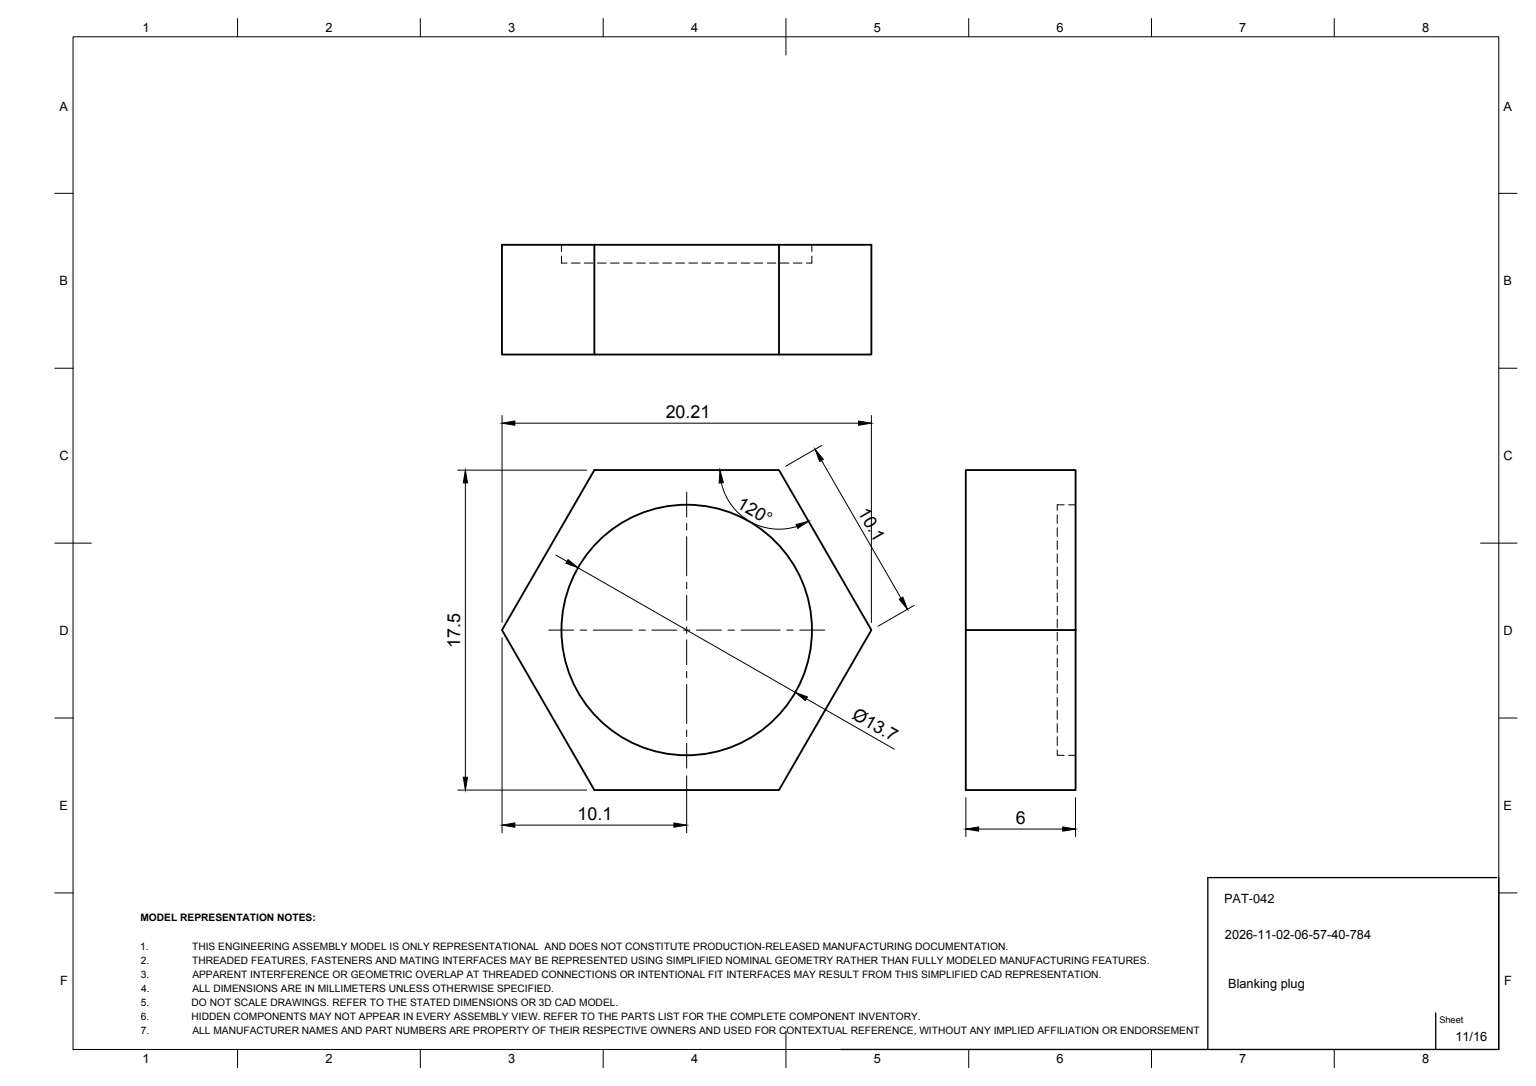
ISO-10303-21;
HEADER;
/* Generated by software containing ST-Developer
 * from STEP Tools, Inc. (www.steptools.com) 
 */

FILE_DESCRIPTION(
/* description */ ('Manifold and mounting hardware'),
/* implementation_level */ '2;1');

FILE_NAME(
/* name */ 'Blanking plug.step',
/* time_stamp */ '2026-10-28T21:46:49-07:00',
/* author */ (''),
/* organization */ (''),
/* preprocessor_version */ 'ST-DEVELOPER v20.2',
/* originating_system */ 'Autodesk Translation Framework v15.17.0.0',
/* authorisation */ '');

FILE_SCHEMA (('AUTOMOTIVE_DESIGN { 1 0 10303 214 3 1 1 }'));
ENDSEC;

DATA;
#10=MECHANICAL_DESIGN_GEOMETRIC_PRESENTATION_REPRESENTATION('',(#158),#5638);
#130=SHAPE_REPRESENTATION_RELATIONSHIP('SRR','None',#5709,#144);
#144=ADVANCED_BREP_SHAPE_REPRESENTATION('',(#172),#5631);
#158=STYLED_ITEM('',(#5874),#172);
#172=MANIFOLD_SOLID_BREP('Body1',#3148);
#240=FACE_BOUND('',#714,.T.);
#317=CYLINDRICAL_SURFACE('',#3559,0.685);
#463=FACE_OUTER_BOUND('',#711,.T.);
#464=FACE_OUTER_BOUND('',#712,.T.);
#465=FACE_OUTER_BOUND('',#713,.T.);
#466=FACE_OUTER_BOUND('',#715,.T.);
#467=FACE_OUTER_BOUND('',#716,.T.);
#468=FACE_OUTER_BOUND('',#717,.T.);
#469=FACE_OUTER_BOUND('',#718,.T.);
#470=FACE_OUTER_BOUND('',#719,.T.);
#471=FACE_OUTER_BOUND('',#720,.T.);
#472=FACE_OUTER_BOUND('',#721,.T.);
#711=EDGE_LOOP('',(#2632,#2633,#2634,#2635));
#712=EDGE_LOOP('',(#2636));
#713=EDGE_LOOP('',(#2637,#2638,#2639,#2640,#2641,#2642));
#714=EDGE_LOOP('',(#2643));
#715=EDGE_LOOP('',(#2644,#2645,#2646,#2647));
#716=EDGE_LOOP('',(#2648,#2649,#2650,#2651));
#717=EDGE_LOOP('',(#2652,#2653,#2654,#2655));
#718=EDGE_LOOP('',(#2656,#2657,#2658,#2659));
#719=EDGE_LOOP('',(#2660,#2661,#2662,#2663));
#720=EDGE_LOOP('',(#2664,#2665,#2666,#2667));
#721=EDGE_LOOP('',(#2668,#2669,#2670,#2671,#2672,#2673));
#868=CIRCLE('',#3560,0.685);
#869=CIRCLE('',#3561,0.685);
#1080=LINE('',#5349,#1327);
#1081=LINE('',#5355,#1328);
#1082=LINE('',#5357,#1329);
#1083=LINE('',#5359,#1330);
#1084=LINE('',#5361,#1331);
#1085=LINE('',#5363,#1332);
#1086=LINE('',#5364,#1333);
#1087=LINE('',#5367,#1334);
#1088=LINE('',#5369,#1335);
#1089=LINE('',#5370,#1336);
#1090=LINE('',#5373,#1337);
#1091=LINE('',#5374,#1338);
#1092=LINE('',#5377,#1339);
#1093=LINE('',#5378,#1340);
#1094=LINE('',#5381,#1341);
#1095=LINE('',#5382,#1342);
#1096=LINE('',#5385,#1343);
#1097=LINE('',#5386,#1344);
#1098=LINE('',#5388,#1345);
#1327=VECTOR('',#4359,0.685);
#1328=VECTOR('',#4366,1.);
#1329=VECTOR('',#4367,1.);
#1330=VECTOR('',#4368,1.);
#1331=VECTOR('',#4369,1.);
#1332=VECTOR('',#4370,1.);
#1333=VECTOR('',#4371,1.);
#1334=VECTOR('',#4374,1.);
#1335=VECTOR('',#4375,1.);
#1336=VECTOR('',#4376,1.);
#1337=VECTOR('',#4379,1.);
#1338=VECTOR('',#4380,1.);
#1339=VECTOR('',#4383,1.);
#1340=VECTOR('',#4384,1.);
#1341=VECTOR('',#4387,1.);
#1342=VECTOR('',#4388,1.);
#1343=VECTOR('',#4391,1.);
#1344=VECTOR('',#4392,1.);
#1345=VECTOR('',#4395,1.);
#1586=VERTEX_POINT('',#5346);
#1587=VERTEX_POINT('',#5348);
#1588=VERTEX_POINT('',#5353);
#1589=VERTEX_POINT('',#5354);
#1590=VERTEX_POINT('',#5356);
#1591=VERTEX_POINT('',#5358);
#1592=VERTEX_POINT('',#5360);
#1593=VERTEX_POINT('',#5362);
#1594=VERTEX_POINT('',#5366);
#1595=VERTEX_POINT('',#5368);
#1596=VERTEX_POINT('',#5372);
#1597=VERTEX_POINT('',#5376);
#1598=VERTEX_POINT('',#5380);
#1599=VERTEX_POINT('',#5384);
#1945=EDGE_CURVE('',#1586,#1586,#868,.T.);
#1946=EDGE_CURVE('',#1586,#1587,#1080,.T.);
#1947=EDGE_CURVE('',#1587,#1587,#869,.T.);
#1948=EDGE_CURVE('',#1588,#1589,#1081,.T.);
#1949=EDGE_CURVE('',#1590,#1588,#1082,.T.);
#1950=EDGE_CURVE('',#1591,#1590,#1083,.T.);
#1951=EDGE_CURVE('',#1592,#1591,#1084,.T.);
#1952=EDGE_CURVE('',#1593,#1592,#1085,.T.);
#1953=EDGE_CURVE('',#1589,#1593,#1086,.T.);
#1954=EDGE_CURVE('',#1588,#1594,#1087,.T.);
#1955=EDGE_CURVE('',#1595,#1594,#1088,.T.);
#1956=EDGE_CURVE('',#1590,#1595,#1089,.T.);
#1957=EDGE_CURVE('',#1596,#1595,#1090,.T.);
#1958=EDGE_CURVE('',#1591,#1596,#1091,.T.);
#1959=EDGE_CURVE('',#1597,#1596,#1092,.T.);
#1960=EDGE_CURVE('',#1592,#1597,#1093,.T.);
#1961=EDGE_CURVE('',#1598,#1597,#1094,.T.);
#1962=EDGE_CURVE('',#1593,#1598,#1095,.T.);
#1963=EDGE_CURVE('',#1599,#1598,#1096,.T.);
#1964=EDGE_CURVE('',#1589,#1599,#1097,.T.);
#1965=EDGE_CURVE('',#1594,#1599,#1098,.T.);
#2632=ORIENTED_EDGE('',*,*,#1945,.F.);
#2633=ORIENTED_EDGE('',*,*,#1946,.T.);
#2634=ORIENTED_EDGE('',*,*,#1947,.T.);
#2635=ORIENTED_EDGE('',*,*,#1946,.F.);
#2636=ORIENTED_EDGE('',*,*,#1947,.F.);
#2637=ORIENTED_EDGE('',*,*,#1948,.F.);
#2638=ORIENTED_EDGE('',*,*,#1949,.F.);
#2639=ORIENTED_EDGE('',*,*,#1950,.F.);
#2640=ORIENTED_EDGE('',*,*,#1951,.F.);
#2641=ORIENTED_EDGE('',*,*,#1952,.F.);
#2642=ORIENTED_EDGE('',*,*,#1953,.F.);
#2643=ORIENTED_EDGE('',*,*,#1945,.T.);
#2644=ORIENTED_EDGE('',*,*,#1949,.T.);
#2645=ORIENTED_EDGE('',*,*,#1954,.T.);
#2646=ORIENTED_EDGE('',*,*,#1955,.F.);
#2647=ORIENTED_EDGE('',*,*,#1956,.F.);
#2648=ORIENTED_EDGE('',*,*,#1950,.T.);
#2649=ORIENTED_EDGE('',*,*,#1956,.T.);
#2650=ORIENTED_EDGE('',*,*,#1957,.F.);
#2651=ORIENTED_EDGE('',*,*,#1958,.F.);
#2652=ORIENTED_EDGE('',*,*,#1951,.T.);
#2653=ORIENTED_EDGE('',*,*,#1958,.T.);
#2654=ORIENTED_EDGE('',*,*,#1959,.F.);
#2655=ORIENTED_EDGE('',*,*,#1960,.F.);
#2656=ORIENTED_EDGE('',*,*,#1952,.T.);
#2657=ORIENTED_EDGE('',*,*,#1960,.T.);
#2658=ORIENTED_EDGE('',*,*,#1961,.F.);
#2659=ORIENTED_EDGE('',*,*,#1962,.F.);
#2660=ORIENTED_EDGE('',*,*,#1953,.T.);
#2661=ORIENTED_EDGE('',*,*,#1962,.T.);
#2662=ORIENTED_EDGE('',*,*,#1963,.F.);
#2663=ORIENTED_EDGE('',*,*,#1964,.F.);
#2664=ORIENTED_EDGE('',*,*,#1948,.T.);
#2665=ORIENTED_EDGE('',*,*,#1964,.T.);
#2666=ORIENTED_EDGE('',*,*,#1965,.F.);
#2667=ORIENTED_EDGE('',*,*,#1954,.F.);
#2668=ORIENTED_EDGE('',*,*,#1965,.T.);
#2669=ORIENTED_EDGE('',*,*,#1963,.T.);
#2670=ORIENTED_EDGE('',*,*,#1961,.T.);
#2671=ORIENTED_EDGE('',*,*,#1959,.T.);
#2672=ORIENTED_EDGE('',*,*,#1957,.T.);
#2673=ORIENTED_EDGE('',*,*,#1955,.T.);
#2918=PLANE('',#3562);
#2919=PLANE('',#3563);
#2920=PLANE('',#3564);
#2921=PLANE('',#3565);
#2922=PLANE('',#3566);
#2923=PLANE('',#3567);
#2924=PLANE('',#3568);
#2925=PLANE('',#3569);
#2926=PLANE('',#3570);
#3087=ADVANCED_FACE('',(#463),#317,.F.);
#3088=ADVANCED_FACE('',(#464),#2918,.F.);
#3089=ADVANCED_FACE('',(#465,#240),#2919,.F.);
#3090=ADVANCED_FACE('',(#466),#2920,.T.);
#3091=ADVANCED_FACE('',(#467),#2921,.T.);
#3092=ADVANCED_FACE('',(#468),#2922,.T.);
#3093=ADVANCED_FACE('',(#469),#2923,.T.);
#3094=ADVANCED_FACE('',(#470),#2924,.T.);
#3095=ADVANCED_FACE('',(#471),#2925,.T.);
#3096=ADVANCED_FACE('',(#472),#2926,.T.);
#3148=CLOSED_SHELL('',(#3087,#3088,#3089,#3090,#3091,#3092,#3093,#3094,
#3095,#3096));
#3558=AXIS2_PLACEMENT_3D('',#5344,#4353,#4354);
#3559=AXIS2_PLACEMENT_3D('',#5345,#4355,#4356);
#3560=AXIS2_PLACEMENT_3D('',#5347,#4357,#4358);
#3561=AXIS2_PLACEMENT_3D('',#5350,#4360,#4361);
#3562=AXIS2_PLACEMENT_3D('',#5351,#4362,#4363);
#3563=AXIS2_PLACEMENT_3D('',#5352,#4364,#4365);
#3564=AXIS2_PLACEMENT_3D('',#5365,#4372,#4373);
#3565=AXIS2_PLACEMENT_3D('',#5371,#4377,#4378);
#3566=AXIS2_PLACEMENT_3D('',#5375,#4381,#4382);
#3567=AXIS2_PLACEMENT_3D('',#5379,#4385,#4386);
#3568=AXIS2_PLACEMENT_3D('',#5383,#4389,#4390);
#3569=AXIS2_PLACEMENT_3D('',#5387,#4393,#4394);
#3570=AXIS2_PLACEMENT_3D('',#5389,#4396,#4397);
#4353=DIRECTION('axis',(0.,0.,1.));
#4354=DIRECTION('refdir',(1.,0.,0.));
#4355=DIRECTION('center_axis',(1.,0.,0.));
#4356=DIRECTION('ref_axis',(0.,0.,-1.));
#4357=DIRECTION('center_axis',(1.,0.,0.));
#4358=DIRECTION('ref_axis',(0.,0.,-1.));
#4359=DIRECTION('',(1.,0.,0.));
#4360=DIRECTION('center_axis',(1.,0.,0.));
#4361=DIRECTION('ref_axis',(0.,0.,-1.));
#4362=DIRECTION('center_axis',(1.,0.,0.));
#4363=DIRECTION('ref_axis',(0.,0.,-1.));
#4364=DIRECTION('center_axis',(1.,0.,0.));
#4365=DIRECTION('ref_axis',(0.,0.,-1.));
#4366=DIRECTION('',(0.,0.5,0.866025403784439));
#4367=DIRECTION('',(0.,1.,-4.39534328316243E-16));
#4368=DIRECTION('',(0.,0.5,-0.866025403784439));
#4369=DIRECTION('',(0.,-0.5,-0.866025403784439));
#4370=DIRECTION('',(0.,-1.,0.));
#4371=DIRECTION('',(0.,-0.5,0.866025403784439));
#4372=DIRECTION('center_axis',(0.,-4.39534328316243E-16,-1.));
#4373=DIRECTION('ref_axis',(0.,1.,-4.39534328316243E-16));
#4374=DIRECTION('',(1.,0.,0.));
#4375=DIRECTION('',(0.,1.,-4.39534328316243E-16));
#4376=DIRECTION('',(1.,0.,0.));
#4377=DIRECTION('center_axis',(0.,-0.866025403784439,-0.5));
#4378=DIRECTION('ref_axis',(0.,0.5,-0.866025403784439));
#4379=DIRECTION('',(0.,0.5,-0.866025403784439));
#4380=DIRECTION('',(1.,0.,0.));
#4381=DIRECTION('center_axis',(0.,-0.866025403784439,0.5));
#4382=DIRECTION('ref_axis',(0.,-0.5,-0.866025403784439));
#4383=DIRECTION('',(0.,-0.5,-0.866025403784439));
#4384=DIRECTION('',(1.,0.,0.));
#4385=DIRECTION('center_axis',(0.,0.,1.));
#4386=DIRECTION('ref_axis',(0.,-1.,0.));
#4387=DIRECTION('',(0.,-1.,0.));
#4388=DIRECTION('',(1.,0.,0.));
#4389=DIRECTION('center_axis',(0.,0.866025403784439,0.5));
#4390=DIRECTION('ref_axis',(0.,-0.5,0.866025403784439));
#4391=DIRECTION('',(0.,-0.5,0.866025403784439));
#4392=DIRECTION('',(1.,0.,0.));
#4393=DIRECTION('center_axis',(0.,0.866025403784439,-0.5));
#4394=DIRECTION('ref_axis',(0.,0.5,0.866025403784439));
#4395=DIRECTION('',(0.,0.5,0.866025403784439));
#4396=DIRECTION('center_axis',(1.,0.,0.));
#4397=DIRECTION('ref_axis',(0.,0.,-1.));
#5344=CARTESIAN_POINT('',(0.,0.,0.));
#5345=CARTESIAN_POINT('Origin',(4.1,0.,3.5));
#5346=CARTESIAN_POINT('',(5.5,-8.38883057415937E-17,4.185));
#5347=CARTESIAN_POINT('Origin',(5.5,0.,3.5));
#5348=CARTESIAN_POINT('',(5.6,-8.38883057415937E-17,4.185));
#5349=CARTESIAN_POINT('',(4.1,-8.38883057415937E-17,4.185));
#5350=CARTESIAN_POINT('Origin',(5.6,0.,3.5));
#5351=CARTESIAN_POINT('Origin',(5.6,0.,3.5));
#5352=CARTESIAN_POINT('Origin',(5.5,0.,3.5));
#5353=CARTESIAN_POINT('',(5.5,0.505181485540923,2.625));
#5354=CARTESIAN_POINT('',(5.5,1.01036297108185,3.5));
#5355=CARTESIAN_POINT('',(5.5,0.505181485540923,2.625));
#5356=CARTESIAN_POINT('',(5.5,-0.505181485540923,2.625));
#5357=CARTESIAN_POINT('',(5.5,-0.505181485540923,2.625));
#5358=CARTESIAN_POINT('',(5.5,-1.01036297108185,3.5));
#5359=CARTESIAN_POINT('',(5.5,-1.01036297108185,3.5));
#5360=CARTESIAN_POINT('',(5.5,-0.505181485540922,4.375));
#5361=CARTESIAN_POINT('',(5.5,-0.505181485540922,4.375));
#5362=CARTESIAN_POINT('',(5.5,0.505181485540923,4.375));
#5363=CARTESIAN_POINT('',(5.5,0.505181485540923,4.375));
#5364=CARTESIAN_POINT('',(5.5,1.01036297108185,3.5));
#5365=CARTESIAN_POINT('Origin',(5.5,-0.505181485540923,2.625));
#5366=CARTESIAN_POINT('',(6.1,0.505181485540923,2.625));
#5367=CARTESIAN_POINT('',(5.5,0.505181485540923,2.625));
#5368=CARTESIAN_POINT('',(6.1,-0.505181485540923,2.625));
#5369=CARTESIAN_POINT('',(6.1,-0.505181485540923,2.625));
#5370=CARTESIAN_POINT('',(5.5,-0.505181485540923,2.625));
#5371=CARTESIAN_POINT('Origin',(5.5,-1.01036297108185,3.5));
#5372=CARTESIAN_POINT('',(6.1,-1.01036297108185,3.5));
#5373=CARTESIAN_POINT('',(6.1,-1.01036297108185,3.5));
#5374=CARTESIAN_POINT('',(5.5,-1.01036297108185,3.5));
#5375=CARTESIAN_POINT('Origin',(5.5,-0.505181485540922,4.375));
#5376=CARTESIAN_POINT('',(6.1,-0.505181485540922,4.375));
#5377=CARTESIAN_POINT('',(6.1,-0.505181485540922,4.375));
#5378=CARTESIAN_POINT('',(5.5,-0.505181485540922,4.375));
#5379=CARTESIAN_POINT('Origin',(5.5,0.505181485540923,4.375));
#5380=CARTESIAN_POINT('',(6.1,0.505181485540923,4.375));
#5381=CARTESIAN_POINT('',(6.1,0.505181485540923,4.375));
#5382=CARTESIAN_POINT('',(5.5,0.505181485540923,4.375));
#5383=CARTESIAN_POINT('Origin',(5.5,1.01036297108185,3.5));
#5384=CARTESIAN_POINT('',(6.1,1.01036297108185,3.5));
#5385=CARTESIAN_POINT('',(6.1,1.01036297108185,3.5));
#5386=CARTESIAN_POINT('',(5.5,1.01036297108185,3.5));
#5387=CARTESIAN_POINT('Origin',(5.5,0.505181485540923,2.625));
#5388=CARTESIAN_POINT('',(6.1,0.505181485540923,2.625));
#5389=CARTESIAN_POINT('Origin',(6.1,0.,3.5));
#5614=UNCERTAINTY_MEASURE_WITH_UNIT(LENGTH_MEASURE(0.001),#5639,
'DISTANCE_ACCURACY_VALUE',
'Maximum model space distance between geometric entities at asserted c
onnectivities');
#5621=UNCERTAINTY_MEASURE_WITH_UNIT(LENGTH_MEASURE(0.001),#5639,
'DISTANCE_ACCURACY_VALUE',
'Maximum model space distance between geometric entities at asserted c
onnectivities');
#5631=(
GEOMETRIC_REPRESENTATION_CONTEXT(3)
GLOBAL_UNCERTAINTY_ASSIGNED_CONTEXT((#5614))
GLOBAL_UNIT_ASSIGNED_CONTEXT((#5639,#5641,#5642))
REPRESENTATION_CONTEXT('','3D')
);
#5638=(
GEOMETRIC_REPRESENTATION_CONTEXT(3)
GLOBAL_UNCERTAINTY_ASSIGNED_CONTEXT((#5621))
GLOBAL_UNIT_ASSIGNED_CONTEXT((#5639,#5641,#5642))
REPRESENTATION_CONTEXT('','3D')
);
#5639=(
LENGTH_UNIT()
NAMED_UNIT(*)
SI_UNIT(.CENTI.,.METRE.)
);
#5641=(
NAMED_UNIT(*)
PLANE_ANGLE_UNIT()
SI_UNIT($,.RADIAN.)
);
#5642=(
NAMED_UNIT(*)
SI_UNIT($,.STERADIAN.)
SOLID_ANGLE_UNIT()
);
#5652=SHAPE_DEFINITION_REPRESENTATION(#5668,#5709);
#5668=PRODUCT_DEFINITION_SHAPE('',$,#5726);
#5709=SHAPE_REPRESENTATION('',(#3558),#5631);
#5716=PRODUCT_DEFINITION_CONTEXT('part definition',#5766,'design');
#5726=PRODUCT_DEFINITION('Blanking plug','Blanking plug',#5742,
#5716);
#5742=PRODUCT_DEFINITION_FORMATION('',$,#5777);
#5766=APPLICATION_CONTEXT(
'Core Data for Automotive Mechanical Design Process');
#5767=PRODUCT_CONTEXT('part definition',#5766,'mechanical');
#5777=PRODUCT('Blanking plug','Blanking plug',
'Blanking plug',(#5767));
#5868=COLOUR_RGB('Off White',0.89,0.88,0.83);
#5869=FILL_AREA_STYLE_COLOUR('',#5868);
#5870=FILL_AREA_STYLE('',(#5869));
#5871=SURFACE_STYLE_FILL_AREA(#5870);
#5872=SURFACE_SIDE_STYLE('',(#5871));
#5873=SURFACE_STYLE_USAGE(.BOTH.,#5872);
#5874=PRESENTATION_STYLE_ASSIGNMENT((#5873));
ENDSEC;
END-ISO-10303-21;
